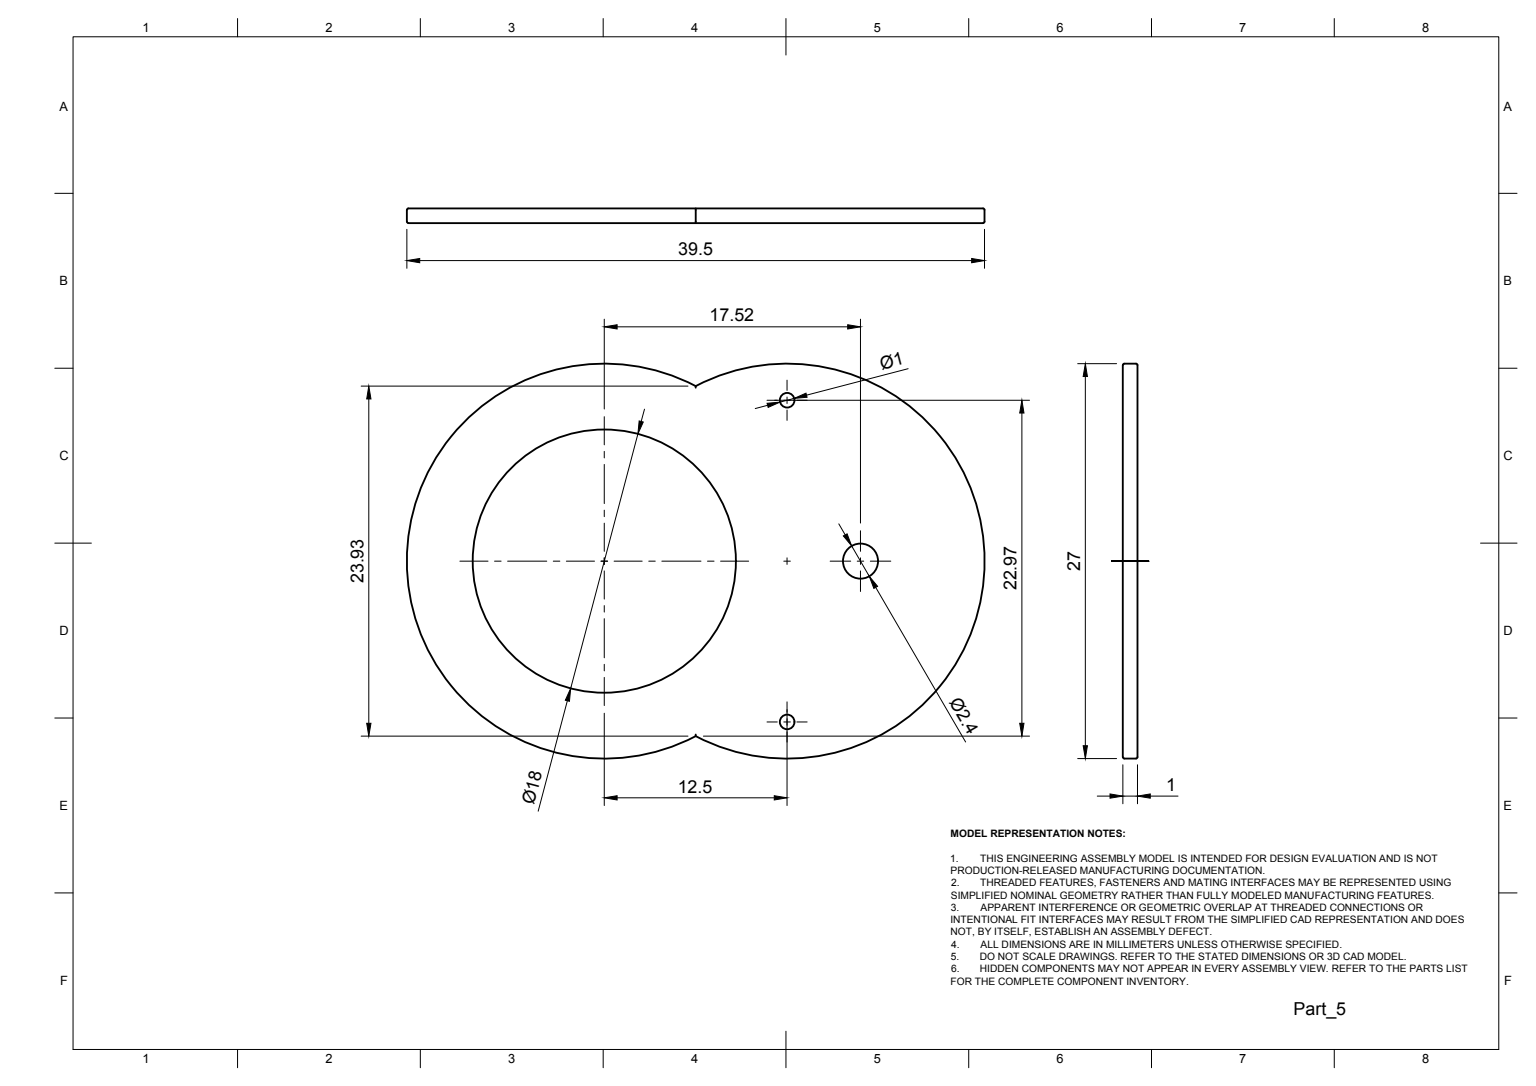
ISO-10303-21;
HEADER;
/* Generated by software containing ST-Developer
 * from STEP Tools, Inc. (www.steptools.com) 
 */

FILE_DESCRIPTION(
/* description */ ('STEP AP242 Edition 2'),
/* implementation_level */ '2;1');

FILE_NAME(
/* name */ 'Part_5.step',
/* time_stamp */ '2026-10-06T10:11:12-07:00',
/* author */ (''),
/* organization */ (''),
/* preprocessor_version */ 'ST-DEVELOPER v20.2',
/* originating_system */ 'Autodesk Translation Framework v15.15.0.0',
/* authorisation */ '');

FILE_SCHEMA (('AUTOMOTIVE_DESIGN { 1 0 10303 214 3 1 1 }'));
ENDSEC;

DATA;
#10=MECHANICAL_DESIGN_GEOMETRIC_PRESENTATION_REPRESENTATION('',(#1797),#54580);
#261=TOROIDAL_SURFACE('',#19179,0.0134,0.0001);
#262=TOROIDAL_SURFACE('',#19180,0.0134,0.0001);
#263=TOROIDAL_SURFACE('',#19181,0.0091,0.0001);
#264=TOROIDAL_SURFACE('',#19183,0.0013,0.0001);
#265=TOROIDAL_SURFACE('',#19185,0.0006,0.0001);
#266=TOROIDAL_SURFACE('',#19187,0.0006,0.0001);
#267=TOROIDAL_SURFACE('',#19189,0.0134,0.0001);
#268=TOROIDAL_SURFACE('',#19190,0.0134,0.0001);
#269=TOROIDAL_SURFACE('',#19191,0.0091,0.0001);
#270=TOROIDAL_SURFACE('',#19193,0.0013,0.0001);
#271=TOROIDAL_SURFACE('',#19195,0.0006,0.0001);
#272=TOROIDAL_SURFACE('',#19197,0.0006,0.0001);
#1348=B_SPLINE_CURVE_WITH_KNOTS('',3,(#48811,#48812,#48813,#48814,#48815,
#48816,#48817,#48818,#48819,#48820,#48821,#48822,#48823,#48824),
 .UNSPECIFIED.,.F.,.F.,(4,2,2,2,2,2,4),(-0.0166502448320504,-0.0131502648660712,
-0.00944645224428793,-0.0052854765179261,-0.00265904695122474,0.,0.000159874250087339),
 .UNSPECIFIED.);
#1349=B_SPLINE_CURVE_WITH_KNOTS('',3,(#48825,#48826,#48827,#48828,#48829,
#48830,#48831,#48832,#48833,#48834,#48835,#48836,#48837,#48838),
 .UNSPECIFIED.,.F.,.F.,(4,2,2,2,2,2,4),(0.0166502448320816,0.0201502247980731,
0.0238540374198661,0.0280150131462326,0.0306414427129375,0.0333004896641681,
0.0334603639142559),.UNSPECIFIED.);
#1350=B_SPLINE_CURVE_WITH_KNOTS('',3,(#48849,#48850,#48851,#48852,#48853,
#48854,#48855,#48856,#48857,#48858,#48859,#48860,#48861,#48862),
 .UNSPECIFIED.,.F.,.F.,(4,2,2,2,2,2,4),(0.016650244832051,0.0201502247980302,
0.0238540374198133,0.0280150131461748,0.0306414427128761,0.0333004896641017,
0.033460363914188),.UNSPECIFIED.);
#1351=B_SPLINE_CURVE_WITH_KNOTS('',3,(#48863,#48864,#48865,#48866,#48867,
#48868,#48869,#48870,#48871,#48872,#48873,#48874,#48875,#48876),
 .UNSPECIFIED.,.F.,.F.,(4,2,2,2,2,2,4),(-0.0166502448320804,-0.0131502648660892,
-0.00944645224429652,-0.00528547651792783,-0.00265904695122334,0.,0.000159874250087547),
 .UNSPECIFIED.);
#1753=SHAPE_REPRESENTATION_RELATIONSHIP('SRR','None',#54640,#1767);
#1767=ADVANCED_BREP_SHAPE_REPRESENTATION('',(#1811),#54576);
#1797=STYLED_ITEM('',(#54712),#1811);
#1811=MANIFOLD_SOLID_BREP('Body1',#17676);
#2305=LINE('',#48735,#2898);
#2306=LINE('',#48739,#2899);
#2307=LINE('',#48776,#2900);
#2308=LINE('',#48786,#2901);
#2309=LINE('',#48796,#2902);
#2310=LINE('',#48806,#2903);
#2898=VECTOR('',#22701,1.);
#2899=VECTOR('',#22704,1.);
#2900=VECTOR('',#22747,0.009);
#2901=VECTOR('',#22758,0.0012);
#2902=VECTOR('',#22769,0.0005);
#2903=VECTOR('',#22780,0.0005);
#3402=CYLINDRICAL_SURFACE('',#19139,0.0135);
#3403=CYLINDRICAL_SURFACE('',#19142,0.0135);
#3404=CYLINDRICAL_SURFACE('',#19159,0.009);
#3405=CYLINDRICAL_SURFACE('',#19164,0.0012);
#3406=CYLINDRICAL_SURFACE('',#19169,0.0005);
#3407=CYLINDRICAL_SURFACE('',#19174,0.0005);
#3514=FACE_BOUND('',#5375,.T.);
#3515=FACE_BOUND('',#5376,.T.);
#3516=FACE_BOUND('',#5377,.T.);
#3517=FACE_BOUND('',#5378,.T.);
#3518=FACE_BOUND('',#5380,.T.);
#3519=FACE_BOUND('',#5381,.T.);
#3520=FACE_BOUND('',#5382,.T.);
#3521=FACE_BOUND('',#5383,.T.);
#4329=FACE_OUTER_BOUND('',#5372,.T.);
#4330=FACE_OUTER_BOUND('',#5373,.T.);
#4331=FACE_OUTER_BOUND('',#5374,.T.);
#4332=FACE_OUTER_BOUND('',#5379,.T.);
#4333=FACE_OUTER_BOUND('',#5384,.T.);
#4334=FACE_OUTER_BOUND('',#5385,.T.);
#4335=FACE_OUTER_BOUND('',#5386,.T.);
#4336=FACE_OUTER_BOUND('',#5387,.T.);
#4337=FACE_OUTER_BOUND('',#5388,.T.);
#4338=FACE_OUTER_BOUND('',#5389,.T.);
#4339=FACE_OUTER_BOUND('',#5390,.T.);
#4340=FACE_OUTER_BOUND('',#5391,.T.);
#4341=FACE_OUTER_BOUND('',#5392,.T.);
#4342=FACE_OUTER_BOUND('',#5393,.T.);
#4343=FACE_OUTER_BOUND('',#5394,.T.);
#4344=FACE_OUTER_BOUND('',#5395,.T.);
#4345=FACE_OUTER_BOUND('',#5396,.T.);
#4346=FACE_OUTER_BOUND('',#5397,.T.);
#4347=FACE_OUTER_BOUND('',#5398,.T.);
#4348=FACE_OUTER_BOUND('',#5399,.T.);
#5372=EDGE_LOOP('',(#15471,#15472,#15473,#15474));
#5373=EDGE_LOOP('',(#15475,#15476,#15477,#15478));
#5374=EDGE_LOOP('',(#15479,#15480));
#5375=EDGE_LOOP('',(#15481));
#5376=EDGE_LOOP('',(#15482));
#5377=EDGE_LOOP('',(#15483));
#5378=EDGE_LOOP('',(#15484));
#5379=EDGE_LOOP('',(#15485,#15486));
#5380=EDGE_LOOP('',(#15487));
#5381=EDGE_LOOP('',(#15488));
#5382=EDGE_LOOP('',(#15489));
#5383=EDGE_LOOP('',(#15490));
#5384=EDGE_LOOP('',(#15491,#15492,#15493,#15494,#15495,#15496));
#5385=EDGE_LOOP('',(#15497,#15498,#15499,#15500,#15501,#15502));
#5386=EDGE_LOOP('',(#15503,#15504,#15505,#15506,#15507,#15508));
#5387=EDGE_LOOP('',(#15509,#15510,#15511,#15512,#15513,#15514));
#5388=EDGE_LOOP('',(#15515,#15516,#15517,#15518));
#5389=EDGE_LOOP('',(#15519,#15520,#15521,#15522));
#5390=EDGE_LOOP('',(#15523,#15524,#15525,#15526,#15527));
#5391=EDGE_LOOP('',(#15528,#15529,#15530,#15531,#15532));
#5392=EDGE_LOOP('',(#15533,#15534,#15535,#15536,#15537));
#5393=EDGE_LOOP('',(#15538,#15539,#15540,#15541,#15542));
#5394=EDGE_LOOP('',(#15543,#15544,#15545,#15546));
#5395=EDGE_LOOP('',(#15547,#15548,#15549,#15550));
#5396=EDGE_LOOP('',(#15551,#15552,#15553,#15554,#15555));
#5397=EDGE_LOOP('',(#15556,#15557,#15558,#15559,#15560));
#5398=EDGE_LOOP('',(#15561,#15562,#15563,#15564,#15565));
#5399=EDGE_LOOP('',(#15566,#15567,#15568,#15569,#15570));
#6272=CIRCLE('',#19140,0.0135);
#6273=CIRCLE('',#19141,0.0135);
#6274=CIRCLE('',#19143,0.0135);
#6275=CIRCLE('',#19144,0.0135);
#6276=CIRCLE('',#19146,0.0134);
#6277=CIRCLE('',#19147,0.0134);
#6278=CIRCLE('',#19148,0.0091);
#6279=CIRCLE('',#19149,0.0013);
#6280=CIRCLE('',#19150,0.0006);
#6281=CIRCLE('',#19151,0.0006);
#6282=CIRCLE('',#19153,0.0134);
#6283=CIRCLE('',#19154,0.0134);
#6284=CIRCLE('',#19155,0.0091);
#6285=CIRCLE('',#19156,0.0013);
#6286=CIRCLE('',#19157,0.0006);
#6287=CIRCLE('',#19158,0.0006);
#6288=CIRCLE('',#19160,0.009);
#6289=CIRCLE('',#19161,0.009);
#6290=CIRCLE('',#19162,0.009);
#6291=CIRCLE('',#19163,0.009);
#6292=CIRCLE('',#19165,0.0012);
#6293=CIRCLE('',#19166,0.0012);
#6294=CIRCLE('',#19167,0.0012);
#6295=CIRCLE('',#19168,0.0012);
#6296=CIRCLE('',#19170,0.0005);
#6297=CIRCLE('',#19171,0.0005);
#6298=CIRCLE('',#19172,0.0005);
#6299=CIRCLE('',#19173,0.0005);
#6300=CIRCLE('',#19175,0.0005);
#6301=CIRCLE('',#19176,0.0005);
#6302=CIRCLE('',#19177,0.0005);
#6303=CIRCLE('',#19178,0.0005);
#6304=CIRCLE('',#19182,0.0001);
#6305=CIRCLE('',#19184,0.0001);
#6306=CIRCLE('',#19186,0.0001);
#6307=CIRCLE('',#19188,0.0001);
#6308=CIRCLE('',#19192,0.0001);
#6309=CIRCLE('',#19194,0.0001);
#6310=CIRCLE('',#19196,0.0001);
#6311=CIRCLE('',#19198,0.0001);
#7989=VERTEX_POINT('',#48733);
#7990=VERTEX_POINT('',#48734);
#7991=VERTEX_POINT('',#48736);
#7992=VERTEX_POINT('',#48738);
#7993=VERTEX_POINT('',#48745);
#7994=VERTEX_POINT('',#48746);
#7995=VERTEX_POINT('',#48749);
#7996=VERTEX_POINT('',#48751);
#7997=VERTEX_POINT('',#48753);
#7998=VERTEX_POINT('',#48755);
#7999=VERTEX_POINT('',#48758);
#8000=VERTEX_POINT('',#48759);
#8001=VERTEX_POINT('',#48762);
#8002=VERTEX_POINT('',#48764);
#8003=VERTEX_POINT('',#48766);
#8004=VERTEX_POINT('',#48768);
#8005=VERTEX_POINT('',#48771);
#8006=VERTEX_POINT('',#48772);
#8007=VERTEX_POINT('',#48775);
#8008=VERTEX_POINT('',#48777);
#8009=VERTEX_POINT('',#48781);
#8010=VERTEX_POINT('',#48782);
#8011=VERTEX_POINT('',#48785);
#8012=VERTEX_POINT('',#48787);
#8013=VERTEX_POINT('',#48791);
#8014=VERTEX_POINT('',#48792);
#8015=VERTEX_POINT('',#48795);
#8016=VERTEX_POINT('',#48797);
#8017=VERTEX_POINT('',#48801);
#8018=VERTEX_POINT('',#48802);
#8019=VERTEX_POINT('',#48805);
#8020=VERTEX_POINT('',#48807);
#10527=EDGE_CURVE('',#7989,#7990,#2305,.T.);
#10528=EDGE_CURVE('',#7990,#7991,#6272,.T.);
#10529=EDGE_CURVE('',#7992,#7991,#2306,.T.);
#10530=EDGE_CURVE('',#7992,#7989,#6273,.F.);
#10531=EDGE_CURVE('',#7991,#7990,#6274,.T.);
#10532=EDGE_CURVE('',#7989,#7992,#6275,.F.);
#10533=EDGE_CURVE('',#7993,#7994,#6276,.T.);
#10534=EDGE_CURVE('',#7994,#7993,#6277,.T.);
#10535=EDGE_CURVE('',#7995,#7995,#6278,.F.);
#10536=EDGE_CURVE('',#7996,#7996,#6279,.F.);
#10537=EDGE_CURVE('',#7997,#7997,#6280,.F.);
#10538=EDGE_CURVE('',#7998,#7998,#6281,.F.);
#10539=EDGE_CURVE('',#7999,#8000,#6282,.F.);
#10540=EDGE_CURVE('',#8000,#7999,#6283,.F.);
#10541=EDGE_CURVE('',#8001,#8001,#6284,.T.);
#10542=EDGE_CURVE('',#8002,#8002,#6285,.T.);
#10543=EDGE_CURVE('',#8003,#8003,#6286,.T.);
#10544=EDGE_CURVE('',#8004,#8004,#6287,.T.);
#10545=EDGE_CURVE('',#8005,#8006,#6288,.T.);
#10546=EDGE_CURVE('',#8006,#8005,#6289,.T.);
#10547=EDGE_CURVE('',#8005,#8007,#2307,.T.);
#10548=EDGE_CURVE('',#8007,#8008,#6290,.F.);
#10549=EDGE_CURVE('',#8008,#8007,#6291,.F.);
#10550=EDGE_CURVE('',#8009,#8010,#6292,.T.);
#10551=EDGE_CURVE('',#8010,#8009,#6293,.T.);
#10552=EDGE_CURVE('',#8009,#8011,#2308,.T.);
#10553=EDGE_CURVE('',#8011,#8012,#6294,.F.);
#10554=EDGE_CURVE('',#8012,#8011,#6295,.F.);
#10555=EDGE_CURVE('',#8013,#8014,#6296,.T.);
#10556=EDGE_CURVE('',#8014,#8013,#6297,.T.);
#10557=EDGE_CURVE('',#8013,#8015,#2309,.T.);
#10558=EDGE_CURVE('',#8015,#8016,#6298,.F.);
#10559=EDGE_CURVE('',#8016,#8015,#6299,.F.);
#10560=EDGE_CURVE('',#8017,#8018,#6300,.T.);
#10561=EDGE_CURVE('',#8018,#8017,#6301,.T.);
#10562=EDGE_CURVE('',#8017,#8019,#2310,.T.);
#10563=EDGE_CURVE('',#8019,#8020,#6302,.F.);
#10564=EDGE_CURVE('',#8020,#8019,#6303,.F.);
#10565=EDGE_CURVE('',#8000,#7990,#1348,.F.);
#10566=EDGE_CURVE('',#7991,#7999,#1349,.T.);
#10567=EDGE_CURVE('',#8001,#8008,#6304,.T.);
#10568=EDGE_CURVE('',#8002,#8012,#6305,.T.);
#10569=EDGE_CURVE('',#8003,#8016,#6306,.T.);
#10570=EDGE_CURVE('',#8004,#8020,#6307,.T.);
#10571=EDGE_CURVE('',#7989,#7993,#1350,.T.);
#10572=EDGE_CURVE('',#7994,#7992,#1351,.F.);
#10573=EDGE_CURVE('',#8006,#7995,#6308,.T.);
#10574=EDGE_CURVE('',#8010,#7996,#6309,.T.);
#10575=EDGE_CURVE('',#8014,#7997,#6310,.T.);
#10576=EDGE_CURVE('',#8018,#7998,#6311,.T.);
#15471=ORIENTED_EDGE('',*,*,#10527,.T.);
#15472=ORIENTED_EDGE('',*,*,#10528,.T.);
#15473=ORIENTED_EDGE('',*,*,#10529,.F.);
#15474=ORIENTED_EDGE('',*,*,#10530,.T.);
#15475=ORIENTED_EDGE('',*,*,#10529,.T.);
#15476=ORIENTED_EDGE('',*,*,#10531,.T.);
#15477=ORIENTED_EDGE('',*,*,#10527,.F.);
#15478=ORIENTED_EDGE('',*,*,#10532,.T.);
#15479=ORIENTED_EDGE('',*,*,#10533,.T.);
#15480=ORIENTED_EDGE('',*,*,#10534,.T.);
#15481=ORIENTED_EDGE('',*,*,#10535,.T.);
#15482=ORIENTED_EDGE('',*,*,#10536,.T.);
#15483=ORIENTED_EDGE('',*,*,#10537,.T.);
#15484=ORIENTED_EDGE('',*,*,#10538,.T.);
#15485=ORIENTED_EDGE('',*,*,#10539,.T.);
#15486=ORIENTED_EDGE('',*,*,#10540,.T.);
#15487=ORIENTED_EDGE('',*,*,#10541,.T.);
#15488=ORIENTED_EDGE('',*,*,#10542,.T.);
#15489=ORIENTED_EDGE('',*,*,#10543,.T.);
#15490=ORIENTED_EDGE('',*,*,#10544,.T.);
#15491=ORIENTED_EDGE('',*,*,#10545,.T.);
#15492=ORIENTED_EDGE('',*,*,#10546,.T.);
#15493=ORIENTED_EDGE('',*,*,#10547,.T.);
#15494=ORIENTED_EDGE('',*,*,#10548,.T.);
#15495=ORIENTED_EDGE('',*,*,#10549,.T.);
#15496=ORIENTED_EDGE('',*,*,#10547,.F.);
#15497=ORIENTED_EDGE('',*,*,#10550,.T.);
#15498=ORIENTED_EDGE('',*,*,#10551,.T.);
#15499=ORIENTED_EDGE('',*,*,#10552,.T.);
#15500=ORIENTED_EDGE('',*,*,#10553,.T.);
#15501=ORIENTED_EDGE('',*,*,#10554,.T.);
#15502=ORIENTED_EDGE('',*,*,#10552,.F.);
#15503=ORIENTED_EDGE('',*,*,#10555,.T.);
#15504=ORIENTED_EDGE('',*,*,#10556,.T.);
#15505=ORIENTED_EDGE('',*,*,#10557,.T.);
#15506=ORIENTED_EDGE('',*,*,#10558,.T.);
#15507=ORIENTED_EDGE('',*,*,#10559,.T.);
#15508=ORIENTED_EDGE('',*,*,#10557,.F.);
#15509=ORIENTED_EDGE('',*,*,#10560,.T.);
#15510=ORIENTED_EDGE('',*,*,#10561,.T.);
#15511=ORIENTED_EDGE('',*,*,#10562,.T.);
#15512=ORIENTED_EDGE('',*,*,#10563,.T.);
#15513=ORIENTED_EDGE('',*,*,#10564,.T.);
#15514=ORIENTED_EDGE('',*,*,#10562,.F.);
#15515=ORIENTED_EDGE('',*,*,#10565,.F.);
#15516=ORIENTED_EDGE('',*,*,#10539,.F.);
#15517=ORIENTED_EDGE('',*,*,#10566,.F.);
#15518=ORIENTED_EDGE('',*,*,#10528,.F.);
#15519=ORIENTED_EDGE('',*,*,#10566,.T.);
#15520=ORIENTED_EDGE('',*,*,#10540,.F.);
#15521=ORIENTED_EDGE('',*,*,#10565,.T.);
#15522=ORIENTED_EDGE('',*,*,#10531,.F.);
#15523=ORIENTED_EDGE('',*,*,#10541,.F.);
#15524=ORIENTED_EDGE('',*,*,#10567,.T.);
#15525=ORIENTED_EDGE('',*,*,#10548,.F.);
#15526=ORIENTED_EDGE('',*,*,#10549,.F.);
#15527=ORIENTED_EDGE('',*,*,#10567,.F.);
#15528=ORIENTED_EDGE('',*,*,#10542,.F.);
#15529=ORIENTED_EDGE('',*,*,#10568,.T.);
#15530=ORIENTED_EDGE('',*,*,#10553,.F.);
#15531=ORIENTED_EDGE('',*,*,#10554,.F.);
#15532=ORIENTED_EDGE('',*,*,#10568,.F.);
#15533=ORIENTED_EDGE('',*,*,#10543,.F.);
#15534=ORIENTED_EDGE('',*,*,#10569,.T.);
#15535=ORIENTED_EDGE('',*,*,#10558,.F.);
#15536=ORIENTED_EDGE('',*,*,#10559,.F.);
#15537=ORIENTED_EDGE('',*,*,#10569,.F.);
#15538=ORIENTED_EDGE('',*,*,#10544,.F.);
#15539=ORIENTED_EDGE('',*,*,#10570,.T.);
#15540=ORIENTED_EDGE('',*,*,#10563,.F.);
#15541=ORIENTED_EDGE('',*,*,#10564,.F.);
#15542=ORIENTED_EDGE('',*,*,#10570,.F.);
#15543=ORIENTED_EDGE('',*,*,#10571,.F.);
#15544=ORIENTED_EDGE('',*,*,#10530,.F.);
#15545=ORIENTED_EDGE('',*,*,#10572,.F.);
#15546=ORIENTED_EDGE('',*,*,#10533,.F.);
#15547=ORIENTED_EDGE('',*,*,#10572,.T.);
#15548=ORIENTED_EDGE('',*,*,#10532,.F.);
#15549=ORIENTED_EDGE('',*,*,#10571,.T.);
#15550=ORIENTED_EDGE('',*,*,#10534,.F.);
#15551=ORIENTED_EDGE('',*,*,#10545,.F.);
#15552=ORIENTED_EDGE('',*,*,#10546,.F.);
#15553=ORIENTED_EDGE('',*,*,#10573,.T.);
#15554=ORIENTED_EDGE('',*,*,#10535,.F.);
#15555=ORIENTED_EDGE('',*,*,#10573,.F.);
#15556=ORIENTED_EDGE('',*,*,#10550,.F.);
#15557=ORIENTED_EDGE('',*,*,#10551,.F.);
#15558=ORIENTED_EDGE('',*,*,#10574,.T.);
#15559=ORIENTED_EDGE('',*,*,#10536,.F.);
#15560=ORIENTED_EDGE('',*,*,#10574,.F.);
#15561=ORIENTED_EDGE('',*,*,#10555,.F.);
#15562=ORIENTED_EDGE('',*,*,#10556,.F.);
#15563=ORIENTED_EDGE('',*,*,#10575,.T.);
#15564=ORIENTED_EDGE('',*,*,#10537,.F.);
#15565=ORIENTED_EDGE('',*,*,#10575,.F.);
#15566=ORIENTED_EDGE('',*,*,#10560,.F.);
#15567=ORIENTED_EDGE('',*,*,#10561,.F.);
#15568=ORIENTED_EDGE('',*,*,#10576,.T.);
#15569=ORIENTED_EDGE('',*,*,#10538,.F.);
#15570=ORIENTED_EDGE('',*,*,#10576,.F.);
#16637=PLANE('',#19145);
#16638=PLANE('',#19152);
#17445=ADVANCED_FACE('',(#4329),#3402,.T.);
#17446=ADVANCED_FACE('',(#4330),#3403,.T.);
#17447=ADVANCED_FACE('',(#4331,#3514,#3515,#3516,#3517),#16637,.T.);
#17448=ADVANCED_FACE('',(#4332,#3518,#3519,#3520,#3521),#16638,.F.);
#17449=ADVANCED_FACE('',(#4333),#3404,.F.);
#17450=ADVANCED_FACE('',(#4334),#3405,.F.);
#17451=ADVANCED_FACE('',(#4335),#3406,.F.);
#17452=ADVANCED_FACE('',(#4336),#3407,.F.);
#17453=ADVANCED_FACE('',(#4337),#261,.T.);
#17454=ADVANCED_FACE('',(#4338),#262,.T.);
#17455=ADVANCED_FACE('',(#4339),#263,.T.);
#17456=ADVANCED_FACE('',(#4340),#264,.T.);
#17457=ADVANCED_FACE('',(#4341),#265,.T.);
#17458=ADVANCED_FACE('',(#4342),#266,.T.);
#17459=ADVANCED_FACE('',(#4343),#267,.T.);
#17460=ADVANCED_FACE('',(#4344),#268,.T.);
#17461=ADVANCED_FACE('',(#4345),#269,.T.);
#17462=ADVANCED_FACE('',(#4346),#270,.T.);
#17463=ADVANCED_FACE('',(#4347),#271,.T.);
#17464=ADVANCED_FACE('',(#4348),#272,.T.);
#17676=CLOSED_SHELL('',(#17445,#17446,#17447,#17448,#17449,#17450,#17451,
#17452,#17453,#17454,#17455,#17456,#17457,#17458,#17459,#17460,#17461,#17462,
#17463,#17464));
#19138=AXIS2_PLACEMENT_3D('',#48731,#22697,#22698);
#19139=AXIS2_PLACEMENT_3D('',#48732,#22699,#22700);
#19140=AXIS2_PLACEMENT_3D('',#48737,#22702,#22703);
#19141=AXIS2_PLACEMENT_3D('',#48740,#22705,#22706);
#19142=AXIS2_PLACEMENT_3D('',#48741,#22707,#22708);
#19143=AXIS2_PLACEMENT_3D('',#48742,#22709,#22710);
#19144=AXIS2_PLACEMENT_3D('',#48743,#22711,#22712);
#19145=AXIS2_PLACEMENT_3D('',#48744,#22713,#22714);
#19146=AXIS2_PLACEMENT_3D('',#48747,#22715,#22716);
#19147=AXIS2_PLACEMENT_3D('',#48748,#22717,#22718);
#19148=AXIS2_PLACEMENT_3D('',#48750,#22719,#22720);
#19149=AXIS2_PLACEMENT_3D('',#48752,#22721,#22722);
#19150=AXIS2_PLACEMENT_3D('',#48754,#22723,#22724);
#19151=AXIS2_PLACEMENT_3D('',#48756,#22725,#22726);
#19152=AXIS2_PLACEMENT_3D('',#48757,#22727,#22728);
#19153=AXIS2_PLACEMENT_3D('',#48760,#22729,#22730);
#19154=AXIS2_PLACEMENT_3D('',#48761,#22731,#22732);
#19155=AXIS2_PLACEMENT_3D('',#48763,#22733,#22734);
#19156=AXIS2_PLACEMENT_3D('',#48765,#22735,#22736);
#19157=AXIS2_PLACEMENT_3D('',#48767,#22737,#22738);
#19158=AXIS2_PLACEMENT_3D('',#48769,#22739,#22740);
#19159=AXIS2_PLACEMENT_3D('',#48770,#22741,#22742);
#19160=AXIS2_PLACEMENT_3D('',#48773,#22743,#22744);
#19161=AXIS2_PLACEMENT_3D('',#48774,#22745,#22746);
#19162=AXIS2_PLACEMENT_3D('',#48778,#22748,#22749);
#19163=AXIS2_PLACEMENT_3D('',#48779,#22750,#22751);
#19164=AXIS2_PLACEMENT_3D('',#48780,#22752,#22753);
#19165=AXIS2_PLACEMENT_3D('',#48783,#22754,#22755);
#19166=AXIS2_PLACEMENT_3D('',#48784,#22756,#22757);
#19167=AXIS2_PLACEMENT_3D('',#48788,#22759,#22760);
#19168=AXIS2_PLACEMENT_3D('',#48789,#22761,#22762);
#19169=AXIS2_PLACEMENT_3D('',#48790,#22763,#22764);
#19170=AXIS2_PLACEMENT_3D('',#48793,#22765,#22766);
#19171=AXIS2_PLACEMENT_3D('',#48794,#22767,#22768);
#19172=AXIS2_PLACEMENT_3D('',#48798,#22770,#22771);
#19173=AXIS2_PLACEMENT_3D('',#48799,#22772,#22773);
#19174=AXIS2_PLACEMENT_3D('',#48800,#22774,#22775);
#19175=AXIS2_PLACEMENT_3D('',#48803,#22776,#22777);
#19176=AXIS2_PLACEMENT_3D('',#48804,#22778,#22779);
#19177=AXIS2_PLACEMENT_3D('',#48808,#22781,#22782);
#19178=AXIS2_PLACEMENT_3D('',#48809,#22783,#22784);
#19179=AXIS2_PLACEMENT_3D('',#48810,#22785,#22786);
#19180=AXIS2_PLACEMENT_3D('',#48839,#22787,#22788);
#19181=AXIS2_PLACEMENT_3D('',#48840,#22789,#22790);
#19182=AXIS2_PLACEMENT_3D('',#48841,#22791,#22792);
#19183=AXIS2_PLACEMENT_3D('',#48842,#22793,#22794);
#19184=AXIS2_PLACEMENT_3D('',#48843,#22795,#22796);
#19185=AXIS2_PLACEMENT_3D('',#48844,#22797,#22798);
#19186=AXIS2_PLACEMENT_3D('',#48845,#22799,#22800);
#19187=AXIS2_PLACEMENT_3D('',#48846,#22801,#22802);
#19188=AXIS2_PLACEMENT_3D('',#48847,#22803,#22804);
#19189=AXIS2_PLACEMENT_3D('',#48848,#22805,#22806);
#19190=AXIS2_PLACEMENT_3D('',#48877,#22807,#22808);
#19191=AXIS2_PLACEMENT_3D('',#48878,#22809,#22810);
#19192=AXIS2_PLACEMENT_3D('',#48879,#22811,#22812);
#19193=AXIS2_PLACEMENT_3D('',#48880,#22813,#22814);
#19194=AXIS2_PLACEMENT_3D('',#48881,#22815,#22816);
#19195=AXIS2_PLACEMENT_3D('',#48882,#22817,#22818);
#19196=AXIS2_PLACEMENT_3D('',#48883,#22819,#22820);
#19197=AXIS2_PLACEMENT_3D('',#48884,#22821,#22822);
#19198=AXIS2_PLACEMENT_3D('',#48885,#22823,#22824);
#22697=DIRECTION('axis',(0.,0.,1.));
#22698=DIRECTION('refdir',(1.,0.,0.));
#22699=DIRECTION('center_axis',(0.,-1.,0.));
#22700=DIRECTION('ref_axis',(-1.,0.,-6.12323399573676E-17));
#22701=DIRECTION('',(0.,-1.,0.));
#22702=DIRECTION('center_axis',(0.,1.,0.));
#22703=DIRECTION('ref_axis',(0.,0.,1.));
#22704=DIRECTION('',(0.,-1.,0.));
#22705=DIRECTION('center_axis',(0.,1.,0.));
#22706=DIRECTION('ref_axis',(0.,0.,1.));
#22707=DIRECTION('center_axis',(0.,-1.,0.));
#22708=DIRECTION('ref_axis',(1.,0.,1.83697019872103E-16));
#22709=DIRECTION('center_axis',(0.,1.,0.));
#22710=DIRECTION('ref_axis',(0.,0.,1.));
#22711=DIRECTION('center_axis',(0.,1.,0.));
#22712=DIRECTION('ref_axis',(0.,0.,1.));
#22713=DIRECTION('center_axis',(0.,1.,0.));
#22714=DIRECTION('ref_axis',(0.,0.,1.));
#22715=DIRECTION('center_axis',(0.,1.,0.));
#22716=DIRECTION('ref_axis',(0.,0.,1.));
#22717=DIRECTION('center_axis',(0.,1.,0.));
#22718=DIRECTION('ref_axis',(0.,0.,1.));
#22719=DIRECTION('center_axis',(0.,1.,0.));
#22720=DIRECTION('ref_axis',(0.,0.,1.));
#22721=DIRECTION('center_axis',(0.,1.,0.));
#22722=DIRECTION('ref_axis',(0.,0.,1.));
#22723=DIRECTION('center_axis',(0.,1.,0.));
#22724=DIRECTION('ref_axis',(0.,0.,1.));
#22725=DIRECTION('center_axis',(0.,1.,0.));
#22726=DIRECTION('ref_axis',(0.,0.,1.));
#22727=DIRECTION('center_axis',(0.,1.,0.));
#22728=DIRECTION('ref_axis',(0.,0.,1.));
#22729=DIRECTION('center_axis',(0.,1.,0.));
#22730=DIRECTION('ref_axis',(0.,0.,1.));
#22731=DIRECTION('center_axis',(0.,1.,0.));
#22732=DIRECTION('ref_axis',(0.,0.,1.));
#22733=DIRECTION('center_axis',(0.,1.,0.));
#22734=DIRECTION('ref_axis',(0.,0.,1.));
#22735=DIRECTION('center_axis',(0.,1.,0.));
#22736=DIRECTION('ref_axis',(0.,0.,1.));
#22737=DIRECTION('center_axis',(0.,1.,0.));
#22738=DIRECTION('ref_axis',(0.,0.,1.));
#22739=DIRECTION('center_axis',(0.,1.,0.));
#22740=DIRECTION('ref_axis',(0.,0.,1.));
#22741=DIRECTION('center_axis',(0.,-1.,0.));
#22742=DIRECTION('ref_axis',(0.,0.,-1.));
#22743=DIRECTION('center_axis',(0.,1.,0.));
#22744=DIRECTION('ref_axis',(0.,0.,1.));
#22745=DIRECTION('center_axis',(0.,1.,0.));
#22746=DIRECTION('ref_axis',(0.,0.,1.));
#22747=DIRECTION('',(0.,-1.,0.));
#22748=DIRECTION('center_axis',(0.,1.,0.));
#22749=DIRECTION('ref_axis',(0.,0.,1.));
#22750=DIRECTION('center_axis',(0.,1.,0.));
#22751=DIRECTION('ref_axis',(0.,0.,1.));
#22752=DIRECTION('center_axis',(0.,-1.,0.));
#22753=DIRECTION('ref_axis',(0.,0.,-1.));
#22754=DIRECTION('center_axis',(0.,1.,0.));
#22755=DIRECTION('ref_axis',(0.,0.,1.));
#22756=DIRECTION('center_axis',(0.,1.,0.));
#22757=DIRECTION('ref_axis',(0.,0.,1.));
#22758=DIRECTION('',(0.,-1.,0.));
#22759=DIRECTION('center_axis',(0.,1.,0.));
#22760=DIRECTION('ref_axis',(0.,0.,1.));
#22761=DIRECTION('center_axis',(0.,1.,0.));
#22762=DIRECTION('ref_axis',(0.,0.,1.));
#22763=DIRECTION('center_axis',(0.,-1.,0.));
#22764=DIRECTION('ref_axis',(0.,0.,-1.));
#22765=DIRECTION('center_axis',(0.,1.,0.));
#22766=DIRECTION('ref_axis',(0.,0.,1.));
#22767=DIRECTION('center_axis',(0.,1.,0.));
#22768=DIRECTION('ref_axis',(0.,0.,1.));
#22769=DIRECTION('',(0.,-1.,0.));
#22770=DIRECTION('center_axis',(0.,1.,0.));
#22771=DIRECTION('ref_axis',(0.,0.,1.));
#22772=DIRECTION('center_axis',(0.,1.,0.));
#22773=DIRECTION('ref_axis',(0.,0.,1.));
#22774=DIRECTION('center_axis',(0.,-1.,0.));
#22775=DIRECTION('ref_axis',(0.,0.,-1.));
#22776=DIRECTION('center_axis',(0.,1.,0.));
#22777=DIRECTION('ref_axis',(0.,0.,1.));
#22778=DIRECTION('center_axis',(0.,1.,0.));
#22779=DIRECTION('ref_axis',(0.,0.,1.));
#22780=DIRECTION('',(0.,-1.,0.));
#22781=DIRECTION('center_axis',(0.,1.,0.));
#22782=DIRECTION('ref_axis',(0.,0.,1.));
#22783=DIRECTION('center_axis',(0.,1.,0.));
#22784=DIRECTION('ref_axis',(0.,0.,1.));
#22785=DIRECTION('center_axis',(0.,1.,0.));
#22786=DIRECTION('ref_axis',(-1.,0.,-1.83697019872103E-16));
#22787=DIRECTION('center_axis',(0.,1.,0.));
#22788=DIRECTION('ref_axis',(1.,0.,-1.60812264967664E-16));
#22789=DIRECTION('center_axis',(0.,1.,0.));
#22790=DIRECTION('ref_axis',(0.,0.,1.));
#22791=DIRECTION('center_axis',(-1.,0.,2.41352831440251E-16));
#22792=DIRECTION('ref_axis',(-2.41352831440251E-16,0.,-1.));
#22793=DIRECTION('center_axis',(0.,1.,0.));
#22794=DIRECTION('ref_axis',(0.,0.,1.));
#22795=DIRECTION('center_axis',(-1.,0.,0.));
#22796=DIRECTION('ref_axis',(0.,0.,-1.));
#22797=DIRECTION('center_axis',(0.,1.,0.));
#22798=DIRECTION('ref_axis',(0.,0.,1.));
#22799=DIRECTION('center_axis',(-1.,0.,1.22464679914735E-16));
#22800=DIRECTION('ref_axis',(-1.22464679914735E-16,0.,-1.));
#22801=DIRECTION('center_axis',(0.,1.,0.));
#22802=DIRECTION('ref_axis',(0.,0.,1.));
#22803=DIRECTION('center_axis',(-1.,0.,1.22464679914735E-16));
#22804=DIRECTION('ref_axis',(-1.22464679914735E-16,0.,-1.));
#22805=DIRECTION('center_axis',(0.,1.,0.));
#22806=DIRECTION('ref_axis',(-1.,0.,-1.83697019872103E-16));
#22807=DIRECTION('center_axis',(0.,1.,0.));
#22808=DIRECTION('ref_axis',(1.,0.,6.12323399573676E-17));
#22809=DIRECTION('center_axis',(0.,1.,0.));
#22810=DIRECTION('ref_axis',(0.,0.,1.));
#22811=DIRECTION('center_axis',(-1.,0.,2.41352831440251E-16));
#22812=DIRECTION('ref_axis',(-2.41352831440251E-16,0.,-1.));
#22813=DIRECTION('center_axis',(0.,1.,0.));
#22814=DIRECTION('ref_axis',(0.,0.,1.));
#22815=DIRECTION('center_axis',(-1.,0.,0.));
#22816=DIRECTION('ref_axis',(0.,0.,-1.));
#22817=DIRECTION('center_axis',(0.,1.,0.));
#22818=DIRECTION('ref_axis',(0.,0.,1.));
#22819=DIRECTION('center_axis',(-1.,0.,1.22464679914735E-16));
#22820=DIRECTION('ref_axis',(-1.22464679914735E-16,0.,-1.));
#22821=DIRECTION('center_axis',(0.,1.,0.));
#22822=DIRECTION('ref_axis',(0.,0.,1.));
#22823=DIRECTION('center_axis',(-1.,0.,1.22464679914735E-16));
#22824=DIRECTION('ref_axis',(-1.22464679914735E-16,0.,-1.));
#48731=CARTESIAN_POINT('',(0.,0.,0.));
#48732=CARTESIAN_POINT('Origin',(0.,0.001,0.));
#48733=CARTESIAN_POINT('',(0.00625,0.0009,-0.0119660979437743));
#48734=CARTESIAN_POINT('',(0.00625,0.0001,-0.0119660979437743));
#48735=CARTESIAN_POINT('',(0.00625,0.001,-0.0119660979437743));
#48736=CARTESIAN_POINT('',(0.00625,0.0001,0.0119660979437743));
#48737=CARTESIAN_POINT('Origin',(0.,0.0001,0.));
#48738=CARTESIAN_POINT('',(0.00625,0.0009,0.0119660979437743));
#48739=CARTESIAN_POINT('',(0.00625,0.001,0.0119660979437743));
#48740=CARTESIAN_POINT('Origin',(0.,0.0009,0.));
#48741=CARTESIAN_POINT('Origin',(0.0125,0.001,-4.59242549680257E-18));
#48742=CARTESIAN_POINT('Origin',(0.0125,0.0001,-4.59242549680257E-18));
#48743=CARTESIAN_POINT('Origin',(0.0125,0.0009,-4.59242549680257E-18));
#48744=CARTESIAN_POINT('Origin',(0.00625,0.001,-2.29621274840129E-18));
#48745=CARTESIAN_POINT('',(0.00625,0.001,-0.0118531641345254));
#48746=CARTESIAN_POINT('',(0.00625,0.001,0.0118531641345254));
#48747=CARTESIAN_POINT('Origin',(0.,0.001,0.));
#48748=CARTESIAN_POINT('Origin',(0.0125,0.001,-4.59242549680257E-18));
#48749=CARTESIAN_POINT('',(0.0125,0.001,-0.00910000000000001));
#48750=CARTESIAN_POINT('Origin',(0.0125,0.001,-4.59242549680257E-18));
#48751=CARTESIAN_POINT('',(-0.00501982557395217,0.001,-0.0013));
#48752=CARTESIAN_POINT('Origin',(-0.00501982557395217,0.001,-2.16840434497101E-19));
#48753=CARTESIAN_POINT('',(-7.34788079488411E-20,0.001,-0.0116));
#48754=CARTESIAN_POINT('Origin',(0.,0.001,-0.011));
#48755=CARTESIAN_POINT('',(-7.34788079488411E-20,0.001,0.0104));
#48756=CARTESIAN_POINT('Origin',(0.,0.001,0.011));
#48757=CARTESIAN_POINT('Origin',(0.00625,0.,-2.29621274840129E-18));
#48758=CARTESIAN_POINT('',(0.00625,0.,0.0118531641345254));
#48759=CARTESIAN_POINT('',(0.00625,0.,-0.0118531641345254));
#48760=CARTESIAN_POINT('Origin',(0.,0.,0.));
#48761=CARTESIAN_POINT('Origin',(0.0125,0.,-4.59242549680257E-18));
#48762=CARTESIAN_POINT('',(0.0125,0.,-0.00910000000000001));
#48763=CARTESIAN_POINT('Origin',(0.0125,0.,-4.59242549680257E-18));
#48764=CARTESIAN_POINT('',(-0.00501982557395217,0.,-0.0013));
#48765=CARTESIAN_POINT('Origin',(-0.00501982557395217,0.,-2.16840434497101E-19));
#48766=CARTESIAN_POINT('',(-7.34788079488411E-20,0.,-0.0116));
#48767=CARTESIAN_POINT('Origin',(0.,0.,-0.011));
#48768=CARTESIAN_POINT('',(-7.34788079488411E-20,0.,0.0104));
#48769=CARTESIAN_POINT('Origin',(0.,0.,0.011));
#48770=CARTESIAN_POINT('Origin',(0.0125,0.0254,-4.59242549680257E-18));
#48771=CARTESIAN_POINT('',(0.0125,0.0009,0.00899999999999999));
#48772=CARTESIAN_POINT('',(0.0125,0.0009,-0.009));
#48773=CARTESIAN_POINT('Origin',(0.0125,0.0009,-4.59242549680257E-18));
#48774=CARTESIAN_POINT('Origin',(0.0125,0.0009,-4.59242549680257E-18));
#48775=CARTESIAN_POINT('',(0.0125,0.0001,0.00899999999999999));
#48776=CARTESIAN_POINT('',(0.0125,0.0254,0.00899999999999999));
#48777=CARTESIAN_POINT('',(0.0125,0.0001,-0.009));
#48778=CARTESIAN_POINT('Origin',(0.0125,0.0001,-4.59242549680257E-18));
#48779=CARTESIAN_POINT('Origin',(0.0125,0.0001,-4.59242549680257E-18));
#48780=CARTESIAN_POINT('Origin',(-0.00501982557395217,0.0254,-2.16840434497101E-19));
#48781=CARTESIAN_POINT('',(-0.00501982557395217,0.0009,0.0012));
#48782=CARTESIAN_POINT('',(-0.00501982557395217,0.0009,-0.0012));
#48783=CARTESIAN_POINT('Origin',(-0.00501982557395217,0.0009,-2.16840434497101E-19));
#48784=CARTESIAN_POINT('Origin',(-0.00501982557395217,0.0009,-2.16840434497101E-19));
#48785=CARTESIAN_POINT('',(-0.00501982557395217,0.0001,0.0012));
#48786=CARTESIAN_POINT('',(-0.00501982557395217,0.0254,0.0012));
#48787=CARTESIAN_POINT('',(-0.00501982557395217,0.0001,-0.0012));
#48788=CARTESIAN_POINT('Origin',(-0.00501982557395217,0.0001,-2.16840434497101E-19));
#48789=CARTESIAN_POINT('Origin',(-0.00501982557395217,0.0001,-2.16840434497101E-19));
#48790=CARTESIAN_POINT('Origin',(0.,0.0254,-0.011));
#48791=CARTESIAN_POINT('',(0.,0.0009,-0.0105));
#48792=CARTESIAN_POINT('',(-6.12323399573675E-20,0.0009,-0.0115));
#48793=CARTESIAN_POINT('Origin',(0.,0.0009,-0.011));
#48794=CARTESIAN_POINT('Origin',(0.,0.0009,-0.011));
#48795=CARTESIAN_POINT('',(0.,0.0001,-0.0105));
#48796=CARTESIAN_POINT('',(-6.12323399573677E-20,0.0254,-0.0105));
#48797=CARTESIAN_POINT('',(-6.12323399573675E-20,0.0001,-0.0115));
#48798=CARTESIAN_POINT('Origin',(0.,0.0001,-0.011));
#48799=CARTESIAN_POINT('Origin',(0.,0.0001,-0.011));
#48800=CARTESIAN_POINT('Origin',(0.,0.0254,0.011));
#48801=CARTESIAN_POINT('',(0.,0.0009,0.0115));
#48802=CARTESIAN_POINT('',(-6.12323399573675E-20,0.0009,0.0105));
#48803=CARTESIAN_POINT('Origin',(0.,0.0009,0.011));
#48804=CARTESIAN_POINT('Origin',(0.,0.0009,0.011));
#48805=CARTESIAN_POINT('',(0.,0.0001,0.0115));
#48806=CARTESIAN_POINT('',(-6.12323399573677E-20,0.0254,0.0115));
#48807=CARTESIAN_POINT('',(-6.12323399573675E-20,0.0001,0.0105));
#48808=CARTESIAN_POINT('Origin',(0.,0.0001,0.011));
#48809=CARTESIAN_POINT('Origin',(0.,0.0001,0.011));
#48810=CARTESIAN_POINT('Origin',(0.,0.0001,0.));
#48811=CARTESIAN_POINT('Ctrl Pts',(0.00624999999999999,0.0001,-0.0119660979437743));
#48812=CARTESIAN_POINT('Ctrl Pts',(0.00624999999999999,8.83792829537417E-5,
-0.0119660979437743));
#48813=CARTESIAN_POINT('Ctrl Pts',(0.00625000000000008,7.69379006756195E-5,
-0.0119638141731892));
#48814=CARTESIAN_POINT('Ctrl Pts',(0.00625000000000009,5.47630188197498E-5,
-0.0119548176774847));
#48815=CARTESIAN_POINT('Ctrl Pts',(0.00625000000004375,4.4420733774185E-5,
-0.0119479855235934));
#48816=CARTESIAN_POINT('Ctrl Pts',(0.00625000000005384,2.54794304335682E-5,
-0.0119299406248958));
#48817=CARTESIAN_POINT('Ctrl Pts',(0.00624999999999999,1.74353766384864E-5,
-0.0119184732907306));
#48818=CARTESIAN_POINT('Ctrl Pts',(0.00624999999999999,7.85927944026424E-6,
-0.0118979845239147));
#48819=CARTESIAN_POINT('Ctrl Pts',(0.00625000000002098,5.03563170544993E-6,
-0.011889655603743));
#48820=CARTESIAN_POINT('Ctrl Pts',(0.00625000000003952,1.15383481991825E-6,
-0.011872472207609));
#48821=CARTESIAN_POINT('Ctrl Pts',(0.00624999999999998,1.2088148348863E-7,
-0.011863625630709));
#48822=CARTESIAN_POINT('Ctrl Pts',(0.00625,3.33322623339041E-9,-0.011854229961993));
#48823=CARTESIAN_POINT('Ctrl Pts',(0.00625,2.88647381170633E-23,-0.0118536970486924));
#48824=CARTESIAN_POINT('Ctrl Pts',(0.00625,0.,-0.0118531641345254));
#48825=CARTESIAN_POINT('Ctrl Pts',(0.00625,0.0001,0.0119660979437743));
#48826=CARTESIAN_POINT('Ctrl Pts',(0.00625,8.83792829537419E-5,0.0119660979437743));
#48827=CARTESIAN_POINT('Ctrl Pts',(0.00625000000000009,7.69379006756203E-5,
0.0119638141731892));
#48828=CARTESIAN_POINT('Ctrl Pts',(0.0062500000000001,5.47630188197589E-5,
0.0119548176774847));
#48829=CARTESIAN_POINT('Ctrl Pts',(0.00625000000004376,4.44207337741988E-5,
0.0119479855235934));
#48830=CARTESIAN_POINT('Ctrl Pts',(0.00625000000005385,2.54794304335679E-5,
0.0119299406248958));
#48831=CARTESIAN_POINT('Ctrl Pts',(0.00625,1.74353766384861E-5,0.0119184732907306));
#48832=CARTESIAN_POINT('Ctrl Pts',(0.00624999999999999,7.85927944026339E-6,
0.0118979845239147));
#48833=CARTESIAN_POINT('Ctrl Pts',(0.00625000000002099,5.03563170544918E-6,
0.011889655603743));
#48834=CARTESIAN_POINT('Ctrl Pts',(0.00625000000003952,1.15383481991727E-6,
0.011872472207609));
#48835=CARTESIAN_POINT('Ctrl Pts',(0.00624999999999998,1.20881483488571E-7,
0.011863625630709));
#48836=CARTESIAN_POINT('Ctrl Pts',(0.00625000000000001,3.33322623339041E-9,
0.011854229961993));
#48837=CARTESIAN_POINT('Ctrl Pts',(0.00625,2.88647381170633E-23,0.0118536970486924));
#48838=CARTESIAN_POINT('Ctrl Pts',(0.00625,0.,0.0118531641345254));
#48839=CARTESIAN_POINT('Origin',(0.0125,0.0001,-4.59242549680257E-18));
#48840=CARTESIAN_POINT('Origin',(0.0125,0.0001,-4.59242549680257E-18));
#48841=CARTESIAN_POINT('Origin',(0.0125,0.0001,-0.00910000000000001));
#48842=CARTESIAN_POINT('Origin',(-0.00501982557395217,0.0001,-2.16840434497101E-19));
#48843=CARTESIAN_POINT('Origin',(-0.00501982557395217,0.0001,-0.0013));
#48844=CARTESIAN_POINT('Origin',(0.,0.0001,-0.011));
#48845=CARTESIAN_POINT('Origin',(-7.34788079488411E-20,0.0001,-0.0116));
#48846=CARTESIAN_POINT('Origin',(0.,0.0001,0.011));
#48847=CARTESIAN_POINT('Origin',(-7.34788079488411E-20,0.0001,0.0104));
#48848=CARTESIAN_POINT('Origin',(0.,0.0009,0.));
#48849=CARTESIAN_POINT('Ctrl Pts',(0.00624999999999999,0.0009,-0.0119660979437743));
#48850=CARTESIAN_POINT('Ctrl Pts',(0.00624999999999999,0.000911620717046258,
-0.0119660979437743));
#48851=CARTESIAN_POINT('Ctrl Pts',(0.00625000000000008,0.00092306209932438,
-0.0119638141731892));
#48852=CARTESIAN_POINT('Ctrl Pts',(0.00625000000000009,0.00094523698118025,
-0.0119548176774847));
#48853=CARTESIAN_POINT('Ctrl Pts',(0.00625000000004375,0.000955579266225815,
-0.0119479855235934));
#48854=CARTESIAN_POINT('Ctrl Pts',(0.00625000000005384,0.000974520569566432,
-0.0119299406248958));
#48855=CARTESIAN_POINT('Ctrl Pts',(0.00624999999999999,0.000982564623361514,
-0.0119184732907306));
#48856=CARTESIAN_POINT('Ctrl Pts',(0.00624999999999999,0.000992140720559736,
-0.0118979845239147));
#48857=CARTESIAN_POINT('Ctrl Pts',(0.00625000000002098,0.00099496436829455,
-0.011889655603743));
#48858=CARTESIAN_POINT('Ctrl Pts',(0.00625000000003952,0.000998846165180082,
-0.011872472207609));
#48859=CARTESIAN_POINT('Ctrl Pts',(0.00624999999999993,0.000999879118516512,
-0.011863625630709));
#48860=CARTESIAN_POINT('Ctrl Pts',(0.00625000000000001,0.000999996666773766,
-0.011854229961993));
#48861=CARTESIAN_POINT('Ctrl Pts',(0.00625,0.001,-0.0118536970486924));
#48862=CARTESIAN_POINT('Ctrl Pts',(0.00625,0.001,-0.0118531641345254));
#48863=CARTESIAN_POINT('Ctrl Pts',(0.00625,0.0009,0.0119660979437743));
#48864=CARTESIAN_POINT('Ctrl Pts',(0.00625,0.000911620717046258,0.0119660979437743));
#48865=CARTESIAN_POINT('Ctrl Pts',(0.00625000000000009,0.00092306209932438,
0.0119638141731892));
#48866=CARTESIAN_POINT('Ctrl Pts',(0.0062500000000001,0.000945236981180241,
0.0119548176774847));
#48867=CARTESIAN_POINT('Ctrl Pts',(0.00625000000004376,0.000955579266225801,
0.0119479855235934));
#48868=CARTESIAN_POINT('Ctrl Pts',(0.00625000000005385,0.000974520569566438,
0.0119299406248958));
#48869=CARTESIAN_POINT('Ctrl Pts',(0.00625,0.00098256462336152,0.0119184732907305));
#48870=CARTESIAN_POINT('Ctrl Pts',(0.00625000000000001,0.00099214072055973,
0.0118979845239147));
#48871=CARTESIAN_POINT('Ctrl Pts',(0.00625000000002099,0.000994964368294546,
0.011889655603743));
#48872=CARTESIAN_POINT('Ctrl Pts',(0.00625000000003952,0.000998846165180083,
0.011872472207609));
#48873=CARTESIAN_POINT('Ctrl Pts',(0.00624999999999998,0.000999879118516511,
0.011863625630709));
#48874=CARTESIAN_POINT('Ctrl Pts',(0.00625000000000001,0.000999996666773767,
0.011854229961993));
#48875=CARTESIAN_POINT('Ctrl Pts',(0.00625,0.001,0.0118536970486924));
#48876=CARTESIAN_POINT('Ctrl Pts',(0.00625,0.001,0.0118531641345254));
#48877=CARTESIAN_POINT('Origin',(0.0125,0.0009,-4.59242549680257E-18));
#48878=CARTESIAN_POINT('Origin',(0.0125,0.0009,-4.59242549680257E-18));
#48879=CARTESIAN_POINT('Origin',(0.0125,0.0009,-0.00910000000000001));
#48880=CARTESIAN_POINT('Origin',(-0.00501982557395217,0.0009,-2.16840434497101E-19));
#48881=CARTESIAN_POINT('Origin',(-0.00501982557395217,0.0009,-0.0013));
#48882=CARTESIAN_POINT('Origin',(0.,0.0009,-0.011));
#48883=CARTESIAN_POINT('Origin',(-7.34788079488411E-20,0.0009,-0.0116));
#48884=CARTESIAN_POINT('Origin',(0.,0.0009,0.011));
#48885=CARTESIAN_POINT('Origin',(-7.34788079488411E-20,0.0009,0.0104));
#54560=UNCERTAINTY_MEASURE_WITH_UNIT(LENGTH_MEASURE(1.E-5),#54581,
'DISTANCE_ACCURACY_VALUE',
'Maximum model space distance between geometric entities at asserted c
onnectivities');
#54564=UNCERTAINTY_MEASURE_WITH_UNIT(LENGTH_MEASURE(1.E-5),#54581,
'DISTANCE_ACCURACY_VALUE',
'Maximum model space distance between geometric entities at asserted c
onnectivities');
#54576=(
GEOMETRIC_REPRESENTATION_CONTEXT(3)
GLOBAL_UNCERTAINTY_ASSIGNED_CONTEXT((#54560))
GLOBAL_UNIT_ASSIGNED_CONTEXT((#54581,#54582,#54583))
REPRESENTATION_CONTEXT('','3D')
);
#54580=(
GEOMETRIC_REPRESENTATION_CONTEXT(3)
GLOBAL_UNCERTAINTY_ASSIGNED_CONTEXT((#54564))
GLOBAL_UNIT_ASSIGNED_CONTEXT((#54581,#54582,#54583))
REPRESENTATION_CONTEXT('','3D')
);
#54581=(
LENGTH_UNIT()
NAMED_UNIT(*)
SI_UNIT($,.METRE.)
);
#54582=(
NAMED_UNIT(*)
PLANE_ANGLE_UNIT()
SI_UNIT($,.RADIAN.)
);
#54583=(
NAMED_UNIT(*)
SI_UNIT($,.STERADIAN.)
SOLID_ANGLE_UNIT()
);
#54595=SHAPE_DEFINITION_REPRESENTATION(#54610,#54640);
#54610=PRODUCT_DEFINITION_SHAPE('',$,#54656);
#54640=SHAPE_REPRESENTATION('',(#19138),#54576);
#54644=PRODUCT_DEFINITION_CONTEXT('part definition',#54691,'design');
#54656=PRODUCT_DEFINITION('Part_5','Part_5',#54671,#54644);
#54671=PRODUCT_DEFINITION_FORMATION('',$,#54704);
#54691=APPLICATION_CONTEXT(
'Core Data for Automotive Mechanical Design Process');
#54692=PRODUCT_CONTEXT('part definition',#54691,'mechanical');
#54704=PRODUCT('Part_5','Part_5','Part 1',(#54692));
#54712=PRESENTATION_STYLE_ASSIGNMENT((#54722));
#54722=SURFACE_STYLE_USAGE(.BOTH.,#54732);
#54732=SURFACE_SIDE_STYLE('',(#54742));
#54742=SURFACE_STYLE_FILL_AREA(#54752);
#54752=FILL_AREA_STYLE('Opaque(26,26,26)',(#54762));
#54762=FILL_AREA_STYLE_COLOUR('Opaque(26,26,26)',#54772);
#54772=COLOUR_RGB('Opaque(26,26,26)', 0.66274510, 0.83137255, 0.94901961);
ENDSEC;
END-ISO-10303-21;
